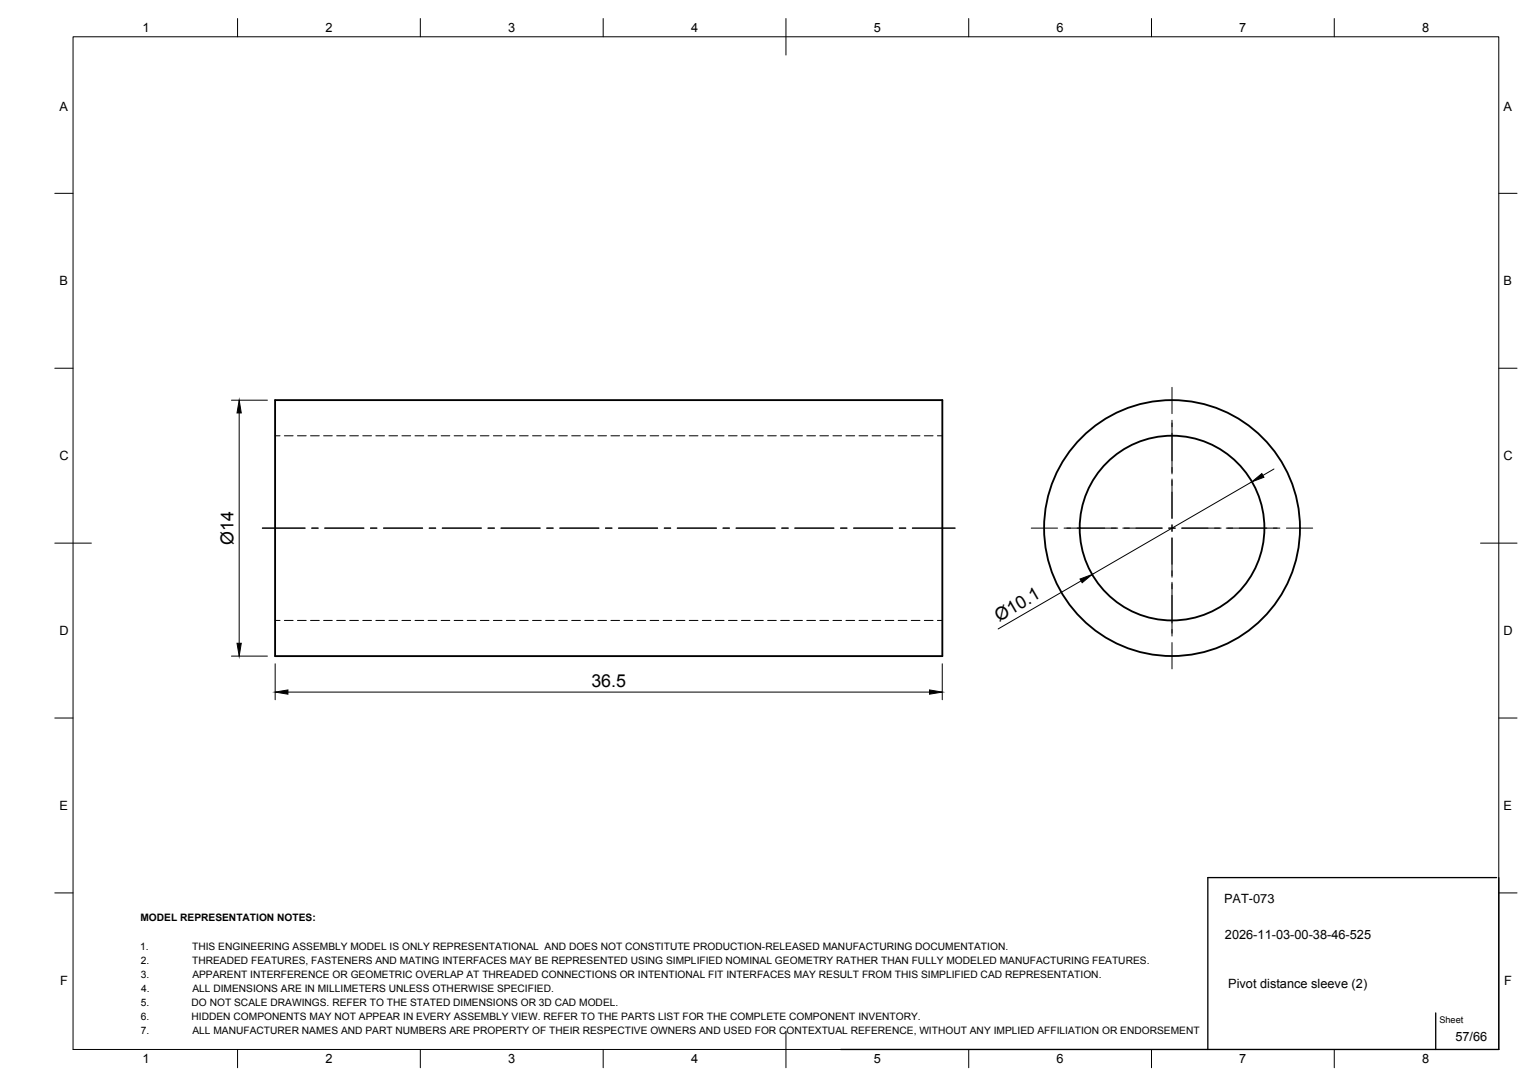
ISO-10303-21;
HEADER;
/* Generated by software containing ST-Developer
 * from STEP Tools, Inc. (www.steptools.com) 
 */

FILE_DESCRIPTION(
/* description */ ('Manual piston pump'),
/* implementation_level */ '2;1');

FILE_NAME(
/* name */ 'Pivot distance sleeve (2).step',
/* time_stamp */ '2026-11-02T16:54:23-08:00',
/* author */ (''),
/* organization */ (''),
/* preprocessor_version */ 'ST-DEVELOPER v20.2',
/* originating_system */ 'Autodesk Translation Framework v15.17.0.0',
/* authorisation */ '');

FILE_SCHEMA (('AUTOMOTIVE_DESIGN { 1 0 10303 214 3 1 1 }'));
ENDSEC;

DATA;
#10=MECHANICAL_DESIGN_GEOMETRIC_PRESENTATION_REPRESENTATION('',(#747),#19043);
#613=SHAPE_REPRESENTATION_RELATIONSHIP('SRR','None',#19363,#676);
#676=ADVANCED_BREP_SHAPE_REPRESENTATION('',(#815),#19030);
#747=STYLED_ITEM('',(#19664),#815);
#815=MANIFOLD_SOLID_BREP('Body1',#9535);
#1024=FACE_BOUND('',#2549,.T.);
#1025=FACE_BOUND('',#2551,.T.);
#1261=CYLINDRICAL_SURFACE('',#11292,0.505000000000001);
#1262=CYLINDRICAL_SURFACE('',#11295,0.699999999999999);
#1774=FACE_OUTER_BOUND('',#2546,.T.);
#1775=FACE_OUTER_BOUND('',#2547,.T.);
#1776=FACE_OUTER_BOUND('',#2548,.T.);
#1777=FACE_OUTER_BOUND('',#2550,.T.);
#2546=EDGE_LOOP('',(#8197,#8198,#8199,#8200));
#2547=EDGE_LOOP('',(#8201,#8202,#8203,#8204));
#2548=EDGE_LOOP('',(#8205));
#2549=EDGE_LOOP('',(#8206));
#2550=EDGE_LOOP('',(#8207));
#2551=EDGE_LOOP('',(#8208));
#3080=CIRCLE('',#11293,0.505000000000001);
#3081=CIRCLE('',#11294,0.505000000000001);
#3082=CIRCLE('',#11296,0.699999999999999);
#3083=CIRCLE('',#11297,0.699999999999999);
#3644=LINE('',#18349,#4248);
#3645=LINE('',#18355,#4249);
#4248=VECTOR('',#14094,0.505000000000001);
#4249=VECTOR('',#14101,0.699999999999999);
#5000=VERTEX_POINT('',#18346);
#5001=VERTEX_POINT('',#18348);
#5002=VERTEX_POINT('',#18352);
#5003=VERTEX_POINT('',#18354);
#6085=EDGE_CURVE('',#5000,#5000,#3080,.T.);
#6086=EDGE_CURVE('',#5000,#5001,#3644,.T.);
#6087=EDGE_CURVE('',#5001,#5001,#3081,.T.);
#6088=EDGE_CURVE('',#5002,#5002,#3082,.T.);
#6089=EDGE_CURVE('',#5002,#5003,#3645,.T.);
#6090=EDGE_CURVE('',#5003,#5003,#3083,.T.);
#8197=ORIENTED_EDGE('',*,*,#6085,.F.);
#8198=ORIENTED_EDGE('',*,*,#6086,.T.);
#8199=ORIENTED_EDGE('',*,*,#6087,.T.);
#8200=ORIENTED_EDGE('',*,*,#6086,.F.);
#8201=ORIENTED_EDGE('',*,*,#6088,.F.);
#8202=ORIENTED_EDGE('',*,*,#6089,.T.);
#8203=ORIENTED_EDGE('',*,*,#6090,.T.);
#8204=ORIENTED_EDGE('',*,*,#6089,.F.);
#8205=ORIENTED_EDGE('',*,*,#6088,.T.);
#8206=ORIENTED_EDGE('',*,*,#6085,.T.);
#8207=ORIENTED_EDGE('',*,*,#6090,.F.);
#8208=ORIENTED_EDGE('',*,*,#6087,.F.);
#8840=PLANE('',#11298);
#8841=PLANE('',#11299);
#9379=ADVANCED_FACE('',(#1774),#1261,.F.);
#9380=ADVANCED_FACE('',(#1775),#1262,.T.);
#9381=ADVANCED_FACE('',(#1776,#1024),#8840,.T.);
#9382=ADVANCED_FACE('',(#1777,#1025),#8841,.F.);
#9535=CLOSED_SHELL('',(#9379,#9380,#9381,#9382));
#11291=AXIS2_PLACEMENT_3D('',#18344,#14088,#14089);
#11292=AXIS2_PLACEMENT_3D('',#18345,#14090,#14091);
#11293=AXIS2_PLACEMENT_3D('',#18347,#14092,#14093);
#11294=AXIS2_PLACEMENT_3D('',#18350,#14095,#14096);
#11295=AXIS2_PLACEMENT_3D('',#18351,#14097,#14098);
#11296=AXIS2_PLACEMENT_3D('',#18353,#14099,#14100);
#11297=AXIS2_PLACEMENT_3D('',#18356,#14102,#14103);
#11298=AXIS2_PLACEMENT_3D('',#18357,#14104,#14105);
#11299=AXIS2_PLACEMENT_3D('',#18358,#14106,#14107);
#14088=DIRECTION('axis',(0.,0.,1.));
#14089=DIRECTION('refdir',(1.,0.,0.));
#14090=DIRECTION('center_axis',(1.,0.,0.));
#14091=DIRECTION('ref_axis',(0.,0.,-1.));
#14092=DIRECTION('center_axis',(-1.,0.,0.));
#14093=DIRECTION('ref_axis',(0.,0.,-1.));
#14094=DIRECTION('',(-1.,0.,0.));
#14095=DIRECTION('center_axis',(-1.,0.,0.));
#14096=DIRECTION('ref_axis',(0.,0.,-1.));
#14097=DIRECTION('center_axis',(1.,0.,0.));
#14098=DIRECTION('ref_axis',(0.,0.,-1.));
#14099=DIRECTION('center_axis',(1.,0.,0.));
#14100=DIRECTION('ref_axis',(0.,0.,-1.));
#14101=DIRECTION('',(-1.,0.,0.));
#14102=DIRECTION('center_axis',(1.,0.,0.));
#14103=DIRECTION('ref_axis',(0.,0.,-1.));
#14104=DIRECTION('center_axis',(1.,0.,0.));
#14105=DIRECTION('ref_axis',(0.,0.,-1.));
#14106=DIRECTION('center_axis',(1.,0.,0.));
#14107=DIRECTION('ref_axis',(0.,0.,-1.));
#18344=CARTESIAN_POINT('',(0.,0.,0.));
#18345=CARTESIAN_POINT('Origin',(-0.6,-4.,10.));
#18346=CARTESIAN_POINT('',(3.05,-4.,10.505));
#18347=CARTESIAN_POINT('Origin',(3.05,-4.,10.));
#18348=CARTESIAN_POINT('',(-0.6,-4.,10.505));
#18349=CARTESIAN_POINT('',(-0.6,-4.,10.505));
#18350=CARTESIAN_POINT('Origin',(-0.6,-4.,10.));
#18351=CARTESIAN_POINT('Origin',(-0.6,-4.,10.));
#18352=CARTESIAN_POINT('',(3.05,-4.,10.7));
#18353=CARTESIAN_POINT('Origin',(3.05,-4.,10.));
#18354=CARTESIAN_POINT('',(-0.6,-4.,10.7));
#18355=CARTESIAN_POINT('',(-0.6,-4.,10.7));
#18356=CARTESIAN_POINT('Origin',(-0.6,-4.,10.));
#18357=CARTESIAN_POINT('Origin',(3.05,-4.,10.));
#18358=CARTESIAN_POINT('Origin',(-0.6,-4.,10.));
#18959=UNCERTAINTY_MEASURE_WITH_UNIT(LENGTH_MEASURE(0.001),#19044,
'DISTANCE_ACCURACY_VALUE',
'Maximum model space distance between geometric entities at asserted c
onnectivities');
#18972=UNCERTAINTY_MEASURE_WITH_UNIT(LENGTH_MEASURE(0.001),#19044,
'DISTANCE_ACCURACY_VALUE',
'Maximum model space distance between geometric entities at asserted c
onnectivities');
#19030=(
GEOMETRIC_REPRESENTATION_CONTEXT(3)
GLOBAL_UNCERTAINTY_ASSIGNED_CONTEXT((#18959))
GLOBAL_UNIT_ASSIGNED_CONTEXT((#19044,#19046,#19047))
REPRESENTATION_CONTEXT('','3D')
);
#19043=(
GEOMETRIC_REPRESENTATION_CONTEXT(3)
GLOBAL_UNCERTAINTY_ASSIGNED_CONTEXT((#18972))
GLOBAL_UNIT_ASSIGNED_CONTEXT((#19044,#19046,#19047))
REPRESENTATION_CONTEXT('','3D')
);
#19044=(
LENGTH_UNIT()
NAMED_UNIT(*)
SI_UNIT(.CENTI.,.METRE.)
);
#19046=(
NAMED_UNIT(*)
PLANE_ANGLE_UNIT()
SI_UNIT($,.RADIAN.)
);
#19047=(
NAMED_UNIT(*)
SI_UNIT($,.STERADIAN.)
SOLID_ANGLE_UNIT()
);
#19105=SHAPE_DEFINITION_REPRESENTATION(#19262,#19363);
#19262=PRODUCT_DEFINITION_SHAPE('',$,#19434);
#19363=SHAPE_REPRESENTATION('',(#11291),#19030);
#19376=PRODUCT_DEFINITION_CONTEXT('part definition',#19588,'design');
#19434=PRODUCT_DEFINITION('2026-11-03-00-38-46-525',
'Pivot distance sleeve (2)',#19504,#19376);
#19504=PRODUCT_DEFINITION_FORMATION('',$,#19647);
#19588=APPLICATION_CONTEXT(
'Core Data for Automotive Mechanical Design Process');
#19589=PRODUCT_CONTEXT('part definition',#19588,'mechanical');
#19647=PRODUCT('2026-11-03-00-38-46-525','Pivot distance sleeve (2)',
'Pivot distance sleeve',(#19589));
#19664=PRESENTATION_STYLE_ASSIGNMENT((#19670));
#19670=SURFACE_STYLE_USAGE(.BOTH.,#19676);
#19676=SURFACE_SIDE_STYLE('',(#19682));
#19682=SURFACE_STYLE_FILL_AREA(#19688);
#19688=FILL_AREA_STYLE('CAD Library Painted - Steel gray',(#19694));
#19694=FILL_AREA_STYLE_COLOUR('CAD Library Painted - Steel gray',#19700);
#19700=COLOUR_RGB('CAD Library Painted - Steel gray',0.592156862745098,
0.631372549019608,0.67843137254902);
ENDSEC;
END-ISO-10303-21;
